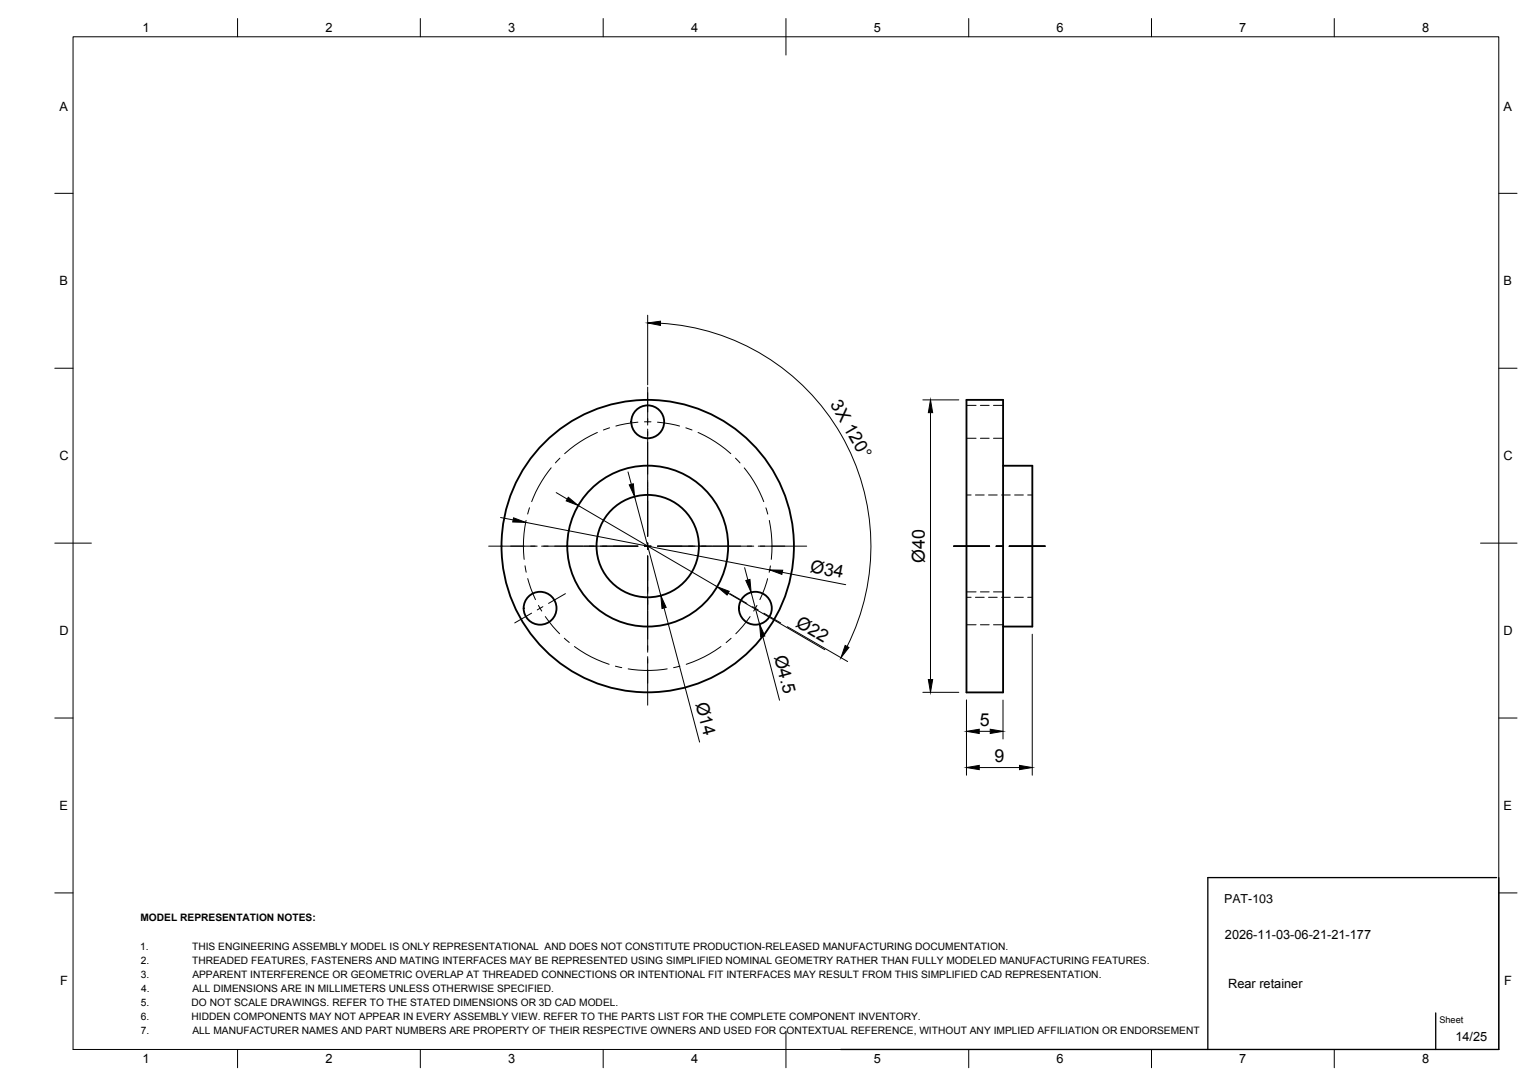
ISO-10303-21;
HEADER;
/* Generated by software containing ST-Developer
 * from STEP Tools, Inc. (www.steptools.com) 
 */

FILE_DESCRIPTION(
/* description */ ('Telescoping shaft support with lock collar'),
/* implementation_level */ '2;1');

FILE_NAME(
/* name */ 'Rear retainer.step',
/* time_stamp */ '2026-10-27T10:48:51-07:00',
/* author */ (''),
/* organization */ (''),
/* preprocessor_version */ 'ST-DEVELOPER v20.2',
/* originating_system */ 'Autodesk Translation Framework v15.17.0.0',
/* authorisation */ '');

FILE_SCHEMA (('AUTOMOTIVE_DESIGN { 1 0 10303 214 3 1 1 }'));
ENDSEC;

DATA;
#10=MECHANICAL_DESIGN_GEOMETRIC_PRESENTATION_REPRESENTATION('',(#250),#7349);
#210=SHAPE_REPRESENTATION_RELATIONSHIP('SRR','None',#7452,#230);
#230=ADVANCED_BREP_SHAPE_REPRESENTATION('',(#270),#7336);
#250=STYLED_ITEM('',(#7620),#270);
#270=MANIFOLD_SOLID_BREP('Body1',#3973);
#319=FACE_BOUND('',#868,.T.);
#320=FACE_BOUND('',#872,.T.);
#321=FACE_BOUND('',#873,.T.);
#322=FACE_BOUND('',#874,.T.);
#323=FACE_BOUND('',#875,.T.);
#324=FACE_BOUND('',#877,.T.);
#325=FACE_BOUND('',#878,.T.);
#326=FACE_BOUND('',#879,.T.);
#327=FACE_BOUND('',#880,.T.);
#421=PLANE('',#4437);
#422=PLANE('',#4444);
#423=PLANE('',#4445);
#597=FACE_OUTER_BOUND('',#863,.T.);
#598=FACE_OUTER_BOUND('',#864,.T.);
#599=FACE_OUTER_BOUND('',#865,.T.);
#600=FACE_OUTER_BOUND('',#866,.T.);
#601=FACE_OUTER_BOUND('',#867,.T.);
#602=FACE_OUTER_BOUND('',#869,.T.);
#603=FACE_OUTER_BOUND('',#870,.T.);
#604=FACE_OUTER_BOUND('',#871,.T.);
#605=FACE_OUTER_BOUND('',#876,.T.);
#863=EDGE_LOOP('',(#3122,#3123,#3124,#3125));
#864=EDGE_LOOP('',(#3126,#3127,#3128,#3129));
#865=EDGE_LOOP('',(#3130,#3131,#3132,#3133));
#866=EDGE_LOOP('',(#3134,#3135,#3136,#3137));
#867=EDGE_LOOP('',(#3138));
#868=EDGE_LOOP('',(#3139));
#869=EDGE_LOOP('',(#3140,#3141,#3142,#3143));
#870=EDGE_LOOP('',(#3144,#3145,#3146,#3147));
#871=EDGE_LOOP('',(#3148));
#872=EDGE_LOOP('',(#3149));
#873=EDGE_LOOP('',(#3150));
#874=EDGE_LOOP('',(#3151));
#875=EDGE_LOOP('',(#3152));
#876=EDGE_LOOP('',(#3153));
#877=EDGE_LOOP('',(#3154));
#878=EDGE_LOOP('',(#3155));
#879=EDGE_LOOP('',(#3156));
#880=EDGE_LOOP('',(#3157));
#1163=LINE('',#6505,#1443);
#1164=LINE('',#6511,#1444);
#1165=LINE('',#6517,#1445);
#1166=LINE('',#6523,#1446);
#1167=LINE('',#6531,#1447);
#1168=LINE('',#6536,#1448);
#1443=VECTOR('',#5283,0.225);
#1444=VECTOR('',#5290,0.225);
#1445=VECTOR('',#5297,0.225);
#1446=VECTOR('',#5304,1.1);
#1447=VECTOR('',#5315,0.7);
#1448=VECTOR('',#5320,2.);
#1691=CIRCLE('',#4426,0.225);
#1692=CIRCLE('',#4427,0.225);
#1693=CIRCLE('',#4429,0.225);
#1694=CIRCLE('',#4430,0.225);
#1695=CIRCLE('',#4432,0.225);
#1696=CIRCLE('',#4433,0.225);
#1697=CIRCLE('',#4435,1.1);
#1698=CIRCLE('',#4436,1.1);
#1699=CIRCLE('',#4438,0.7);
#1700=CIRCLE('',#4440,0.7);
#1701=CIRCLE('',#4442,2.);
#1702=CIRCLE('',#4443,2.);
#1958=VERTEX_POINT('',#6502);
#1959=VERTEX_POINT('',#6504);
#1960=VERTEX_POINT('',#6508);
#1961=VERTEX_POINT('',#6510);
#1962=VERTEX_POINT('',#6514);
#1963=VERTEX_POINT('',#6516);
#1964=VERTEX_POINT('',#6520);
#1965=VERTEX_POINT('',#6522);
#1966=VERTEX_POINT('',#6526);
#1967=VERTEX_POINT('',#6529);
#1968=VERTEX_POINT('',#6533);
#1969=VERTEX_POINT('',#6535);
#2373=EDGE_CURVE('',#1958,#1958,#1691,.T.);
#2374=EDGE_CURVE('',#1958,#1959,#1163,.T.);
#2375=EDGE_CURVE('',#1959,#1959,#1692,.T.);
#2376=EDGE_CURVE('',#1960,#1960,#1693,.T.);
#2377=EDGE_CURVE('',#1960,#1961,#1164,.T.);
#2378=EDGE_CURVE('',#1961,#1961,#1694,.T.);
#2379=EDGE_CURVE('',#1962,#1962,#1695,.T.);
#2380=EDGE_CURVE('',#1962,#1963,#1165,.T.);
#2381=EDGE_CURVE('',#1963,#1963,#1696,.T.);
#2382=EDGE_CURVE('',#1964,#1964,#1697,.T.);
#2383=EDGE_CURVE('',#1964,#1965,#1166,.T.);
#2384=EDGE_CURVE('',#1965,#1965,#1698,.T.);
#2385=EDGE_CURVE('',#1966,#1966,#1699,.T.);
#2386=EDGE_CURVE('',#1967,#1967,#1700,.T.);
#2387=EDGE_CURVE('',#1967,#1966,#1167,.T.);
#2388=EDGE_CURVE('',#1968,#1968,#1701,.T.);
#2389=EDGE_CURVE('',#1968,#1969,#1168,.T.);
#2390=EDGE_CURVE('',#1969,#1969,#1702,.T.);
#3122=ORIENTED_EDGE('',*,*,#2373,.F.);
#3123=ORIENTED_EDGE('',*,*,#2374,.T.);
#3124=ORIENTED_EDGE('',*,*,#2375,.F.);
#3125=ORIENTED_EDGE('',*,*,#2374,.F.);
#3126=ORIENTED_EDGE('',*,*,#2376,.F.);
#3127=ORIENTED_EDGE('',*,*,#2377,.T.);
#3128=ORIENTED_EDGE('',*,*,#2378,.F.);
#3129=ORIENTED_EDGE('',*,*,#2377,.F.);
#3130=ORIENTED_EDGE('',*,*,#2379,.F.);
#3131=ORIENTED_EDGE('',*,*,#2380,.T.);
#3132=ORIENTED_EDGE('',*,*,#2381,.F.);
#3133=ORIENTED_EDGE('',*,*,#2380,.F.);
#3134=ORIENTED_EDGE('',*,*,#2382,.F.);
#3135=ORIENTED_EDGE('',*,*,#2383,.T.);
#3136=ORIENTED_EDGE('',*,*,#2384,.T.);
#3137=ORIENTED_EDGE('',*,*,#2383,.F.);
#3138=ORIENTED_EDGE('',*,*,#2384,.F.);
#3139=ORIENTED_EDGE('',*,*,#2385,.F.);
#3140=ORIENTED_EDGE('',*,*,#2386,.F.);
#3141=ORIENTED_EDGE('',*,*,#2387,.T.);
#3142=ORIENTED_EDGE('',*,*,#2385,.T.);
#3143=ORIENTED_EDGE('',*,*,#2387,.F.);
#3144=ORIENTED_EDGE('',*,*,#2388,.F.);
#3145=ORIENTED_EDGE('',*,*,#2389,.T.);
#3146=ORIENTED_EDGE('',*,*,#2390,.T.);
#3147=ORIENTED_EDGE('',*,*,#2389,.F.);
#3148=ORIENTED_EDGE('',*,*,#2388,.T.);
#3149=ORIENTED_EDGE('',*,*,#2375,.T.);
#3150=ORIENTED_EDGE('',*,*,#2378,.T.);
#3151=ORIENTED_EDGE('',*,*,#2381,.T.);
#3152=ORIENTED_EDGE('',*,*,#2386,.T.);
#3153=ORIENTED_EDGE('',*,*,#2390,.F.);
#3154=ORIENTED_EDGE('',*,*,#2373,.T.);
#3155=ORIENTED_EDGE('',*,*,#2376,.T.);
#3156=ORIENTED_EDGE('',*,*,#2379,.T.);
#3157=ORIENTED_EDGE('',*,*,#2382,.T.);
#3700=CYLINDRICAL_SURFACE('',#4425,0.225);
#3701=CYLINDRICAL_SURFACE('',#4428,0.225);
#3702=CYLINDRICAL_SURFACE('',#4431,0.225);
#3703=CYLINDRICAL_SURFACE('',#4434,1.1);
#3704=CYLINDRICAL_SURFACE('',#4439,0.7);
#3705=CYLINDRICAL_SURFACE('',#4441,2.);
#3840=ADVANCED_FACE('',(#597),#3700,.F.);
#3841=ADVANCED_FACE('',(#598),#3701,.F.);
#3842=ADVANCED_FACE('',(#599),#3702,.F.);
#3843=ADVANCED_FACE('',(#600),#3703,.T.);
#3844=ADVANCED_FACE('',(#601,#319),#421,.F.);
#3845=ADVANCED_FACE('',(#602),#3704,.F.);
#3846=ADVANCED_FACE('',(#603),#3705,.T.);
#3847=ADVANCED_FACE('',(#604,#320,#321,#322,#323),#422,.T.);
#3848=ADVANCED_FACE('',(#605,#324,#325,#326,#327),#423,.F.);
#3973=CLOSED_SHELL('',(#3840,#3841,#3842,#3843,#3844,#3845,#3846,#3847,
#3848));
#4424=AXIS2_PLACEMENT_3D('',#6500,#5277,#5278);
#4425=AXIS2_PLACEMENT_3D('',#6501,#5279,#5280);
#4426=AXIS2_PLACEMENT_3D('',#6503,#5281,#5282);
#4427=AXIS2_PLACEMENT_3D('',#6506,#5284,#5285);
#4428=AXIS2_PLACEMENT_3D('',#6507,#5286,#5287);
#4429=AXIS2_PLACEMENT_3D('',#6509,#5288,#5289);
#4430=AXIS2_PLACEMENT_3D('',#6512,#5291,#5292);
#4431=AXIS2_PLACEMENT_3D('',#6513,#5293,#5294);
#4432=AXIS2_PLACEMENT_3D('',#6515,#5295,#5296);
#4433=AXIS2_PLACEMENT_3D('',#6518,#5298,#5299);
#4434=AXIS2_PLACEMENT_3D('',#6519,#5300,#5301);
#4435=AXIS2_PLACEMENT_3D('',#6521,#5302,#5303);
#4436=AXIS2_PLACEMENT_3D('',#6524,#5305,#5306);
#4437=AXIS2_PLACEMENT_3D('',#6525,#5307,#5308);
#4438=AXIS2_PLACEMENT_3D('',#6527,#5309,#5310);
#4439=AXIS2_PLACEMENT_3D('',#6528,#5311,#5312);
#4440=AXIS2_PLACEMENT_3D('',#6530,#5313,#5314);
#4441=AXIS2_PLACEMENT_3D('',#6532,#5316,#5317);
#4442=AXIS2_PLACEMENT_3D('',#6534,#5318,#5319);
#4443=AXIS2_PLACEMENT_3D('',#6537,#5321,#5322);
#4444=AXIS2_PLACEMENT_3D('',#6538,#5323,#5324);
#4445=AXIS2_PLACEMENT_3D('',#6539,#5325,#5326);
#5277=DIRECTION('axis',(0.,0.,1.));
#5278=DIRECTION('refdir',(1.,0.,0.));
#5279=DIRECTION('center_axis',(1.,0.,0.));
#5280=DIRECTION('ref_axis',(0.,0.,-1.));
#5281=DIRECTION('center_axis',(1.,0.,0.));
#5282=DIRECTION('ref_axis',(0.,0.,-1.));
#5283=DIRECTION('',(1.,0.,0.));
#5284=DIRECTION('center_axis',(-1.,0.,0.));
#5285=DIRECTION('ref_axis',(0.,0.,-1.));
#5286=DIRECTION('center_axis',(1.,0.,0.));
#5287=DIRECTION('ref_axis',(0.,0.,-1.));
#5288=DIRECTION('center_axis',(1.,0.,0.));
#5289=DIRECTION('ref_axis',(0.,0.,-1.));
#5290=DIRECTION('',(1.,0.,0.));
#5291=DIRECTION('center_axis',(-1.,0.,0.));
#5292=DIRECTION('ref_axis',(0.,0.,-1.));
#5293=DIRECTION('center_axis',(1.,0.,0.));
#5294=DIRECTION('ref_axis',(0.,0.,-1.));
#5295=DIRECTION('center_axis',(1.,0.,0.));
#5296=DIRECTION('ref_axis',(0.,0.,-1.));
#5297=DIRECTION('',(1.,0.,0.));
#5298=DIRECTION('center_axis',(-1.,0.,0.));
#5299=DIRECTION('ref_axis',(0.,0.,-1.));
#5300=DIRECTION('center_axis',(1.,0.,0.));
#5301=DIRECTION('ref_axis',(0.,0.,-1.));
#5302=DIRECTION('center_axis',(1.,0.,0.));
#5303=DIRECTION('ref_axis',(0.,0.,-1.));
#5304=DIRECTION('',(-1.,0.,0.));
#5305=DIRECTION('center_axis',(1.,0.,0.));
#5306=DIRECTION('ref_axis',(0.,0.,-1.));
#5307=DIRECTION('center_axis',(1.,0.,0.));
#5308=DIRECTION('ref_axis',(0.,0.,-1.));
#5309=DIRECTION('center_axis',(-1.,0.,0.));
#5310=DIRECTION('ref_axis',(0.,0.,-1.));
#5311=DIRECTION('center_axis',(1.,0.,0.));
#5312=DIRECTION('ref_axis',(0.,0.,-1.));
#5313=DIRECTION('center_axis',(-1.,0.,0.));
#5314=DIRECTION('ref_axis',(0.,0.,-1.));
#5315=DIRECTION('',(-1.,0.,0.));
#5316=DIRECTION('center_axis',(1.,0.,0.));
#5317=DIRECTION('ref_axis',(0.,0.,-1.));
#5318=DIRECTION('center_axis',(1.,0.,0.));
#5319=DIRECTION('ref_axis',(0.,0.,-1.));
#5320=DIRECTION('',(-1.,0.,0.));
#5321=DIRECTION('center_axis',(1.,0.,0.));
#5322=DIRECTION('ref_axis',(0.,0.,-1.));
#5323=DIRECTION('center_axis',(1.,0.,0.));
#5324=DIRECTION('ref_axis',(0.,0.,-1.));
#5325=DIRECTION('center_axis',(1.,0.,0.));
#5326=DIRECTION('ref_axis',(0.,0.,-1.));
#6500=CARTESIAN_POINT('',(0.,0.,0.));
#6501=CARTESIAN_POINT('Origin',(-0.6,1.04094977927525E-16,5.2));
#6502=CARTESIAN_POINT('',(-0.5,7.65404249467096E-17,5.425));
#6503=CARTESIAN_POINT('Origin',(-0.5,1.04094977927525E-16,5.2));
#6504=CARTESIAN_POINT('',(0.,1.3164953090834E-16,5.425));
#6505=CARTESIAN_POINT('',(-0.6,7.65404249467096E-17,5.425));
#6506=CARTESIAN_POINT('Origin',(0.,1.04094977927525E-16,5.2));
#6507=CARTESIAN_POINT('Origin',(-0.6,-1.47224318643355,2.65));
#6508=CARTESIAN_POINT('',(-0.5,-1.47224318643355,2.875));
#6509=CARTESIAN_POINT('Origin',(-0.5,-1.47224318643355,2.65));
#6510=CARTESIAN_POINT('',(0.,-1.47224318643355,2.875));
#6511=CARTESIAN_POINT('',(-0.6,-1.47224318643355,2.875));
#6512=CARTESIAN_POINT('Origin',(0.,-1.47224318643355,2.65));
#6513=CARTESIAN_POINT('Origin',(-0.6,1.47224318643355,2.65));
#6514=CARTESIAN_POINT('',(-0.5,1.47224318643355,2.875));
#6515=CARTESIAN_POINT('Origin',(-0.5,1.47224318643355,2.65));
#6516=CARTESIAN_POINT('',(0.,1.47224318643355,2.875));
#6517=CARTESIAN_POINT('',(-0.6,1.47224318643355,2.875));
#6518=CARTESIAN_POINT('Origin',(0.,1.47224318643355,2.65));
#6519=CARTESIAN_POINT('Origin',(-0.9,0.,3.5));
#6520=CARTESIAN_POINT('',(-0.5,-1.34711147906209E-16,4.6));
#6521=CARTESIAN_POINT('Origin',(-0.5,0.,3.5));
#6522=CARTESIAN_POINT('',(-0.9,-1.34711147906209E-16,4.6));
#6523=CARTESIAN_POINT('',(-0.9,-1.34711147906209E-16,4.6));
#6524=CARTESIAN_POINT('Origin',(-0.9,0.,3.5));
#6525=CARTESIAN_POINT('Origin',(-0.9,0.,3.5));
#6526=CARTESIAN_POINT('',(-0.9,-8.57252759403147E-17,4.2));
#6527=CARTESIAN_POINT('Origin',(-0.9,0.,3.5));
#6528=CARTESIAN_POINT('Origin',(-0.5,0.,3.5));
#6529=CARTESIAN_POINT('',(0.,-8.57252759403147E-17,4.2));
#6530=CARTESIAN_POINT('Origin',(0.,0.,3.5));
#6531=CARTESIAN_POINT('',(-0.5,-8.57252759403147E-17,4.2));
#6532=CARTESIAN_POINT('Origin',(-0.5,0.,3.5));
#6533=CARTESIAN_POINT('',(0.,-2.44929359829471E-16,5.5));
#6534=CARTESIAN_POINT('Origin',(0.,0.,3.5));
#6535=CARTESIAN_POINT('',(-0.5,-2.44929359829471E-16,5.5));
#6536=CARTESIAN_POINT('',(-0.5,-2.44929359829471E-16,5.5));
#6537=CARTESIAN_POINT('Origin',(-0.5,0.,3.5));
#6538=CARTESIAN_POINT('Origin',(0.,0.,3.5));
#6539=CARTESIAN_POINT('Origin',(-0.5,0.,3.5));
#7311=UNCERTAINTY_MEASURE_WITH_UNIT(LENGTH_MEASURE(0.001),#7350,
'DISTANCE_ACCURACY_VALUE',
'Maximum model space distance between geometric entities at asserted c
onnectivities');
#7324=UNCERTAINTY_MEASURE_WITH_UNIT(LENGTH_MEASURE(0.001),#7350,
'DISTANCE_ACCURACY_VALUE',
'Maximum model space distance between geometric entities at asserted c
onnectivities');
#7336=(
GEOMETRIC_REPRESENTATION_CONTEXT(3)
GLOBAL_UNCERTAINTY_ASSIGNED_CONTEXT((#7311))
GLOBAL_UNIT_ASSIGNED_CONTEXT((#7350,#7352,#7353))
REPRESENTATION_CONTEXT('','3D')
);
#7349=(
GEOMETRIC_REPRESENTATION_CONTEXT(3)
GLOBAL_UNCERTAINTY_ASSIGNED_CONTEXT((#7324))
GLOBAL_UNIT_ASSIGNED_CONTEXT((#7350,#7352,#7353))
REPRESENTATION_CONTEXT('','3D')
);
#7350=(
LENGTH_UNIT()
NAMED_UNIT(*)
SI_UNIT(.CENTI.,.METRE.)
);
#7352=(
NAMED_UNIT(*)
PLANE_ANGLE_UNIT()
SI_UNIT($,.RADIAN.)
);
#7353=(
NAMED_UNIT(*)
SI_UNIT($,.STERADIAN.)
SOLID_ANGLE_UNIT()
);
#7365=SHAPE_DEFINITION_REPRESENTATION(#7389,#7452);
#7389=PRODUCT_DEFINITION_SHAPE('',$,#7477);
#7452=SHAPE_REPRESENTATION('',(#4424),#7336);
#7465=PRODUCT_DEFINITION_CONTEXT('part definition',#7539,'design');
#7477=PRODUCT_DEFINITION('Rear retainer','Rear retainer',#7501,#7465);
#7501=PRODUCT_DEFINITION_FORMATION('',$,#7552);
#7539=APPLICATION_CONTEXT(
'Core Data for Automotive Mechanical Design Process');
#7540=PRODUCT_CONTEXT('part definition',#7539,'mechanical');
#7552=PRODUCT('Rear retainer','Rear retainer','Rear retainer',(#7540));
#7614=COLOUR_RGB('Sky Blue',0.24,0.69,0.87);
#7615=FILL_AREA_STYLE_COLOUR('',#7614);
#7616=FILL_AREA_STYLE('',(#7615));
#7617=SURFACE_STYLE_FILL_AREA(#7616);
#7618=SURFACE_SIDE_STYLE('',(#7617));
#7619=SURFACE_STYLE_USAGE(.BOTH.,#7618);
#7620=PRESENTATION_STYLE_ASSIGNMENT((#7619));
ENDSEC;
END-ISO-10303-21;
